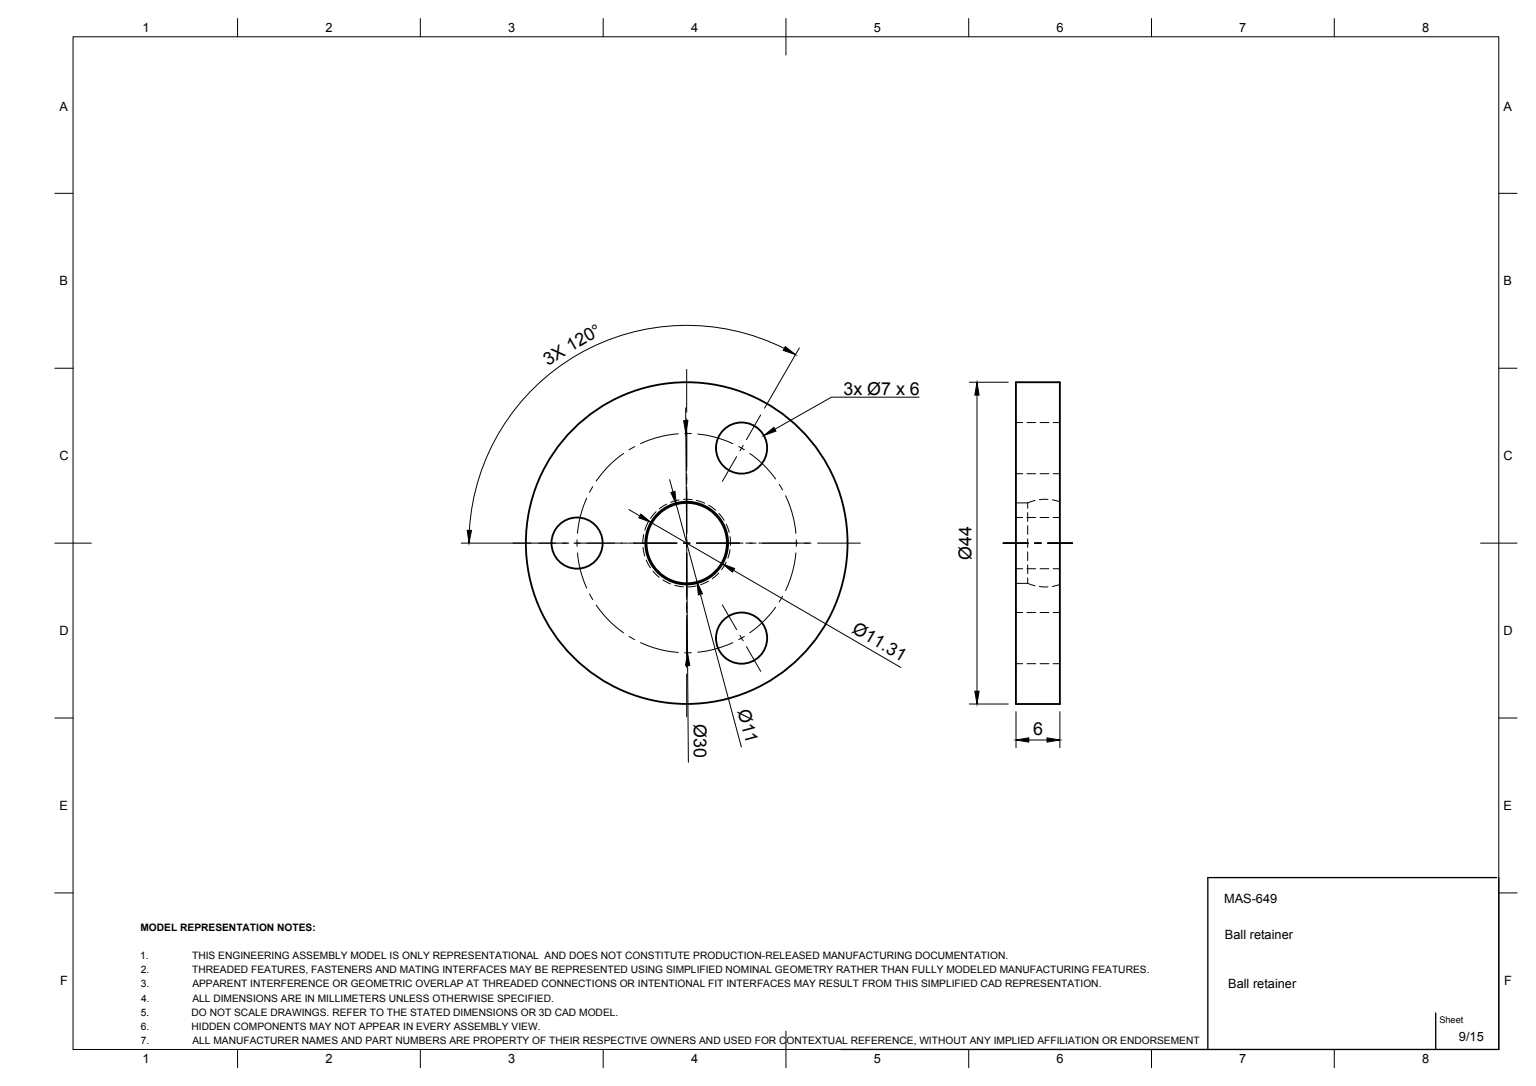
ISO-10303-21;
HEADER;
/* Generated by software containing ST-Developer
 * from STEP Tools, Inc. (www.steptools.com) 
 */

FILE_DESCRIPTION(
/* description */ ('Independent equipment support assembly with bolted 600 x 500 mm welde
d perimeter frame, four adjustable legs and swivel feet. Nominal overa
ll height 518 mm. No load rating assigned.'),
/* implementation_level */ '2;1');

FILE_NAME(
/* name */ 'Ball retainer.step',
/* time_stamp */ '2026-11-07T17:30:39-08:00',
/* author */ (''),
/* organization */ (''),
/* preprocessor_version */ 'ST-DEVELOPER v20.2',
/* originating_system */ 'Autodesk Translation Framework v15.17.0.0',
/* authorisation */ '');

FILE_SCHEMA (('AUTOMOTIVE_DESIGN { 1 0 10303 214 3 1 1 }'));
ENDSEC;

DATA;
#10=MECHANICAL_DESIGN_GEOMETRIC_PRESENTATION_REPRESENTATION('',(#2218),#63755);
#12=SPHERICAL_SURFACE('',#15242,6.);
#449=CIRCLE('',#15234,3.5);
#450=CIRCLE('',#15235,3.5);
#451=CIRCLE('',#15237,3.5);
#452=CIRCLE('',#15238,3.5);
#453=CIRCLE('',#15240,3.5);
#454=CIRCLE('',#15241,3.5);
#455=CIRCLE('',#15243,5.65685424949238);
#456=CIRCLE('',#15244,6.);
#457=CIRCLE('',#15245,5.5);
#458=CIRCLE('',#15247,5.5);
#459=CIRCLE('',#15249,22.);
#460=CIRCLE('',#15250,22.);
#1993=CYLINDRICAL_SURFACE('',#15233,3.5);
#1994=CYLINDRICAL_SURFACE('',#15236,3.5);
#1995=CYLINDRICAL_SURFACE('',#15239,3.5);
#1996=CYLINDRICAL_SURFACE('',#15246,5.5);
#1997=CYLINDRICAL_SURFACE('',#15248,22.);
#2186=SHAPE_REPRESENTATION_RELATIONSHIP('SRR','None',#63871,#2202);
#2202=ADVANCED_BREP_SHAPE_REPRESENTATION('',(#2234),#63749);
#2218=STYLED_ITEM('',(#63959),#2234);
#2234=MANIFOLD_SOLID_BREP('Body1',#14319);
#2285=FACE_BOUND('',#3650,.T.);
#2286=FACE_BOUND('',#3651,.T.);
#2287=FACE_BOUND('',#3652,.T.);
#2288=FACE_BOUND('',#3653,.T.);
#2289=FACE_BOUND('',#3655,.T.);
#2290=FACE_BOUND('',#3656,.T.);
#2291=FACE_BOUND('',#3657,.T.);
#2292=FACE_BOUND('',#3658,.T.);
#2838=FACE_OUTER_BOUND('',#3643,.T.);
#2839=FACE_OUTER_BOUND('',#3644,.T.);
#2840=FACE_OUTER_BOUND('',#3645,.T.);
#2841=FACE_OUTER_BOUND('',#3646,.T.);
#2842=FACE_OUTER_BOUND('',#3647,.T.);
#2843=FACE_OUTER_BOUND('',#3648,.T.);
#2844=FACE_OUTER_BOUND('',#3649,.T.);
#2845=FACE_OUTER_BOUND('',#3654,.T.);
#3643=EDGE_LOOP('',(#12155,#12156,#12157,#12158));
#3644=EDGE_LOOP('',(#12159,#12160,#12161,#12162));
#3645=EDGE_LOOP('',(#12163,#12164,#12165,#12166));
#3646=EDGE_LOOP('',(#12167,#12168,#12169,#12170));
#3647=EDGE_LOOP('',(#12171,#12172,#12173,#12174));
#3648=EDGE_LOOP('',(#12175,#12176,#12177,#12178));
#3649=EDGE_LOOP('',(#12179));
#3650=EDGE_LOOP('',(#12180));
#3651=EDGE_LOOP('',(#12181));
#3652=EDGE_LOOP('',(#12182));
#3653=EDGE_LOOP('',(#12183));
#3654=EDGE_LOOP('',(#12184));
#3655=EDGE_LOOP('',(#12185));
#3656=EDGE_LOOP('',(#12186));
#3657=EDGE_LOOP('',(#12187));
#3658=EDGE_LOOP('',(#12188));
#4490=LINE('',#51513,#5326);
#4491=LINE('',#51519,#5327);
#4492=LINE('',#51525,#5328);
#4493=LINE('',#51536,#5329);
#4494=LINE('',#51541,#5330);
#5326=VECTOR('',#17585,3.5);
#5327=VECTOR('',#17592,3.5);
#5328=VECTOR('',#17599,3.5);
#5329=VECTOR('',#17614,5.5);
#5330=VECTOR('',#17619,22.);
#6568=VERTEX_POINT('',#51510);
#6569=VERTEX_POINT('',#51512);
#6570=VERTEX_POINT('',#51516);
#6571=VERTEX_POINT('',#51518);
#6572=VERTEX_POINT('',#51522);
#6573=VERTEX_POINT('',#51524);
#6574=VERTEX_POINT('',#51528);
#6575=VERTEX_POINT('',#51530);
#6576=VERTEX_POINT('',#51534);
#6577=VERTEX_POINT('',#51538);
#6578=VERTEX_POINT('',#51540);
#8500=EDGE_CURVE('',#6568,#6568,#449,.T.);
#8501=EDGE_CURVE('',#6568,#6569,#4490,.T.);
#8502=EDGE_CURVE('',#6569,#6569,#450,.T.);
#8503=EDGE_CURVE('',#6570,#6570,#451,.T.);
#8504=EDGE_CURVE('',#6570,#6571,#4491,.T.);
#8505=EDGE_CURVE('',#6571,#6571,#452,.T.);
#8506=EDGE_CURVE('',#6572,#6572,#453,.T.);
#8507=EDGE_CURVE('',#6572,#6573,#4492,.T.);
#8508=EDGE_CURVE('',#6573,#6573,#454,.T.);
#8509=EDGE_CURVE('',#6574,#6574,#455,.T.);
#8510=EDGE_CURVE('',#6574,#6575,#456,.T.);
#8511=EDGE_CURVE('',#6575,#6575,#457,.T.);
#8512=EDGE_CURVE('',#6576,#6576,#458,.T.);
#8513=EDGE_CURVE('',#6576,#6575,#4493,.T.);
#8514=EDGE_CURVE('',#6577,#6577,#459,.T.);
#8515=EDGE_CURVE('',#6577,#6578,#4494,.T.);
#8516=EDGE_CURVE('',#6578,#6578,#460,.T.);
#12155=ORIENTED_EDGE('',*,*,#8500,.F.);
#12156=ORIENTED_EDGE('',*,*,#8501,.T.);
#12157=ORIENTED_EDGE('',*,*,#8502,.F.);
#12158=ORIENTED_EDGE('',*,*,#8501,.F.);
#12159=ORIENTED_EDGE('',*,*,#8503,.F.);
#12160=ORIENTED_EDGE('',*,*,#8504,.T.);
#12161=ORIENTED_EDGE('',*,*,#8505,.F.);
#12162=ORIENTED_EDGE('',*,*,#8504,.F.);
#12163=ORIENTED_EDGE('',*,*,#8506,.F.);
#12164=ORIENTED_EDGE('',*,*,#8507,.T.);
#12165=ORIENTED_EDGE('',*,*,#8508,.F.);
#12166=ORIENTED_EDGE('',*,*,#8507,.F.);
#12167=ORIENTED_EDGE('',*,*,#8509,.F.);
#12168=ORIENTED_EDGE('',*,*,#8510,.T.);
#12169=ORIENTED_EDGE('',*,*,#8511,.F.);
#12170=ORIENTED_EDGE('',*,*,#8510,.F.);
#12171=ORIENTED_EDGE('',*,*,#8512,.F.);
#12172=ORIENTED_EDGE('',*,*,#8513,.T.);
#12173=ORIENTED_EDGE('',*,*,#8511,.T.);
#12174=ORIENTED_EDGE('',*,*,#8513,.F.);
#12175=ORIENTED_EDGE('',*,*,#8514,.F.);
#12176=ORIENTED_EDGE('',*,*,#8515,.T.);
#12177=ORIENTED_EDGE('',*,*,#8516,.T.);
#12178=ORIENTED_EDGE('',*,*,#8515,.F.);
#12179=ORIENTED_EDGE('',*,*,#8514,.T.);
#12180=ORIENTED_EDGE('',*,*,#8500,.T.);
#12181=ORIENTED_EDGE('',*,*,#8503,.T.);
#12182=ORIENTED_EDGE('',*,*,#8506,.T.);
#12183=ORIENTED_EDGE('',*,*,#8512,.T.);
#12184=ORIENTED_EDGE('',*,*,#8516,.F.);
#12185=ORIENTED_EDGE('',*,*,#8502,.T.);
#12186=ORIENTED_EDGE('',*,*,#8505,.T.);
#12187=ORIENTED_EDGE('',*,*,#8508,.T.);
#12188=ORIENTED_EDGE('',*,*,#8509,.T.);
#13516=PLANE('',#15251);
#13517=PLANE('',#15252);
#14084=ADVANCED_FACE('',(#2838),#1993,.F.);
#14085=ADVANCED_FACE('',(#2839),#1994,.F.);
#14086=ADVANCED_FACE('',(#2840),#1995,.F.);
#14087=ADVANCED_FACE('',(#2841),#12,.F.);
#14088=ADVANCED_FACE('',(#2842),#1996,.F.);
#14089=ADVANCED_FACE('',(#2843),#1997,.T.);
#14090=ADVANCED_FACE('',(#2844,#2285,#2286,#2287,#2288),#13516,.T.);
#14091=ADVANCED_FACE('',(#2845,#2289,#2290,#2291,#2292),#13517,.F.);
#14319=CLOSED_SHELL('',(#14084,#14085,#14086,#14087,#14088,#14089,#14090,
#14091));
#15232=AXIS2_PLACEMENT_3D('',#51508,#17579,#17580);
#15233=AXIS2_PLACEMENT_3D('',#51509,#17581,#17582);
#15234=AXIS2_PLACEMENT_3D('',#51511,#17583,#17584);
#15235=AXIS2_PLACEMENT_3D('',#51514,#17586,#17587);
#15236=AXIS2_PLACEMENT_3D('',#51515,#17588,#17589);
#15237=AXIS2_PLACEMENT_3D('',#51517,#17590,#17591);
#15238=AXIS2_PLACEMENT_3D('',#51520,#17593,#17594);
#15239=AXIS2_PLACEMENT_3D('',#51521,#17595,#17596);
#15240=AXIS2_PLACEMENT_3D('',#51523,#17597,#17598);
#15241=AXIS2_PLACEMENT_3D('',#51526,#17600,#17601);
#15242=AXIS2_PLACEMENT_3D('',#51527,#17602,#17603);
#15243=AXIS2_PLACEMENT_3D('',#51529,#17604,#17605);
#15244=AXIS2_PLACEMENT_3D('',#51531,#17606,#17607);
#15245=AXIS2_PLACEMENT_3D('',#51532,#17608,#17609);
#15246=AXIS2_PLACEMENT_3D('',#51533,#17610,#17611);
#15247=AXIS2_PLACEMENT_3D('',#51535,#17612,#17613);
#15248=AXIS2_PLACEMENT_3D('',#51537,#17615,#17616);
#15249=AXIS2_PLACEMENT_3D('',#51539,#17617,#17618);
#15250=AXIS2_PLACEMENT_3D('',#51542,#17620,#17621);
#15251=AXIS2_PLACEMENT_3D('',#51543,#17622,#17623);
#15252=AXIS2_PLACEMENT_3D('',#51544,#17624,#17625);
#17579=DIRECTION('axis',(0.,0.,1.));
#17580=DIRECTION('refdir',(1.,0.,0.));
#17581=DIRECTION('center_axis',(0.,0.,-1.));
#17582=DIRECTION('ref_axis',(1.,0.,0.));
#17583=DIRECTION('center_axis',(0.,0.,-1.));
#17584=DIRECTION('ref_axis',(1.,0.,0.));
#17585=DIRECTION('',(0.,0.,-1.));
#17586=DIRECTION('center_axis',(0.,0.,1.));
#17587=DIRECTION('ref_axis',(1.,0.,0.));
#17588=DIRECTION('center_axis',(0.,0.,-1.));
#17589=DIRECTION('ref_axis',(1.,0.,0.));
#17590=DIRECTION('center_axis',(0.,0.,-1.));
#17591=DIRECTION('ref_axis',(1.,0.,0.));
#17592=DIRECTION('',(0.,0.,-1.));
#17593=DIRECTION('center_axis',(0.,0.,1.));
#17594=DIRECTION('ref_axis',(1.,0.,0.));
#17595=DIRECTION('center_axis',(0.,0.,-1.));
#17596=DIRECTION('ref_axis',(1.,0.,0.));
#17597=DIRECTION('center_axis',(0.,0.,-1.));
#17598=DIRECTION('ref_axis',(1.,0.,0.));
#17599=DIRECTION('',(0.,0.,-1.));
#17600=DIRECTION('center_axis',(0.,0.,1.));
#17601=DIRECTION('ref_axis',(1.,0.,0.));
#17602=DIRECTION('center_axis',(6.12323399573677E-17,0.,1.));
#17603=DIRECTION('ref_axis',(1.,0.,0.));
#17604=DIRECTION('center_axis',(0.,0.,1.));
#17605=DIRECTION('ref_axis',(0.,-1.,0.));
#17606=DIRECTION('center_axis',(-1.22464679914735E-16,1.,0.));
#17607=DIRECTION('ref_axis',(-1.,-1.22464679914735E-16,0.));
#17608=DIRECTION('center_axis',(0.,0.,-1.));
#17609=DIRECTION('ref_axis',(1.,0.,0.));
#17610=DIRECTION('center_axis',(0.,0.,1.));
#17611=DIRECTION('ref_axis',(1.,0.,0.));
#17612=DIRECTION('center_axis',(0.,0.,-1.));
#17613=DIRECTION('ref_axis',(1.,0.,0.));
#17614=DIRECTION('',(0.,0.,-1.));
#17615=DIRECTION('center_axis',(0.,0.,1.));
#17616=DIRECTION('ref_axis',(1.,0.,0.));
#17617=DIRECTION('center_axis',(0.,0.,1.));
#17618=DIRECTION('ref_axis',(1.,0.,0.));
#17619=DIRECTION('',(0.,0.,-1.));
#17620=DIRECTION('center_axis',(0.,0.,1.));
#17621=DIRECTION('ref_axis',(1.,0.,0.));
#17622=DIRECTION('center_axis',(0.,0.,1.));
#17623=DIRECTION('ref_axis',(1.,0.,0.));
#17624=DIRECTION('center_axis',(0.,0.,1.));
#17625=DIRECTION('ref_axis',(1.,0.,0.));
#51508=CARTESIAN_POINT('',(0.,0.,0.));
#51509=CARTESIAN_POINT('Origin',(-7.5,12.9903810567666,15.));
#51510=CARTESIAN_POINT('',(-11.,12.9903810567666,18.));
#51511=CARTESIAN_POINT('Origin',(-7.5,12.9903810567666,18.));
#51512=CARTESIAN_POINT('',(-11.,12.9903810567666,12.));
#51513=CARTESIAN_POINT('',(-11.,12.9903810567666,15.));
#51514=CARTESIAN_POINT('Origin',(-7.5,12.9903810567666,12.));
#51515=CARTESIAN_POINT('Origin',(15.,0.,15.));
#51516=CARTESIAN_POINT('',(11.5,4.28626379701574E-16,18.));
#51517=CARTESIAN_POINT('Origin',(15.,0.,18.));
#51518=CARTESIAN_POINT('',(11.5,4.28626379701574E-16,12.));
#51519=CARTESIAN_POINT('',(11.5,4.28626379701574E-16,15.));
#51520=CARTESIAN_POINT('Origin',(15.,0.,12.));
#51521=CARTESIAN_POINT('Origin',(-7.50000000000001,-12.9903810567666,15.));
#51522=CARTESIAN_POINT('',(-11.,-12.9903810567666,18.));
#51523=CARTESIAN_POINT('Origin',(-7.50000000000001,-12.9903810567666,18.));
#51524=CARTESIAN_POINT('',(-11.,-12.9903810567666,12.));
#51525=CARTESIAN_POINT('',(-11.,-12.9903810567666,15.));
#51526=CARTESIAN_POINT('Origin',(-7.50000000000001,-12.9903810567666,12.));
#51527=CARTESIAN_POINT('Origin',(5.55111512312578E-16,0.,14.));
#51528=CARTESIAN_POINT('',(-5.65685424949238,-6.92764844988394E-16,12.));
#51529=CARTESIAN_POINT('Origin',(5.55111512312578E-16,0.,12.));
#51530=CARTESIAN_POINT('',(-5.5,6.73555739531044E-16,16.3979157616564));
#51531=CARTESIAN_POINT('Origin',(5.55111512312578E-16,0.,14.));
#51532=CARTESIAN_POINT('Origin',(0.,0.,16.3979157616564));
#51533=CARTESIAN_POINT('Origin',(0.,0.,12.));
#51534=CARTESIAN_POINT('',(-5.5,-6.73555739531044E-16,18.));
#51535=CARTESIAN_POINT('Origin',(0.,0.,18.));
#51536=CARTESIAN_POINT('',(-5.5,-6.73555739531044E-16,12.));
#51537=CARTESIAN_POINT('Origin',(0.,0.,12.));
#51538=CARTESIAN_POINT('',(-22.,-2.69422295812418E-15,18.));
#51539=CARTESIAN_POINT('Origin',(0.,0.,18.));
#51540=CARTESIAN_POINT('',(-22.,-2.69422295812418E-15,12.));
#51541=CARTESIAN_POINT('',(-22.,-2.69422295812418E-15,12.));
#51542=CARTESIAN_POINT('Origin',(0.,0.,12.));
#51543=CARTESIAN_POINT('Origin',(0.,0.,18.));
#51544=CARTESIAN_POINT('Origin',(0.,0.,12.));
#63729=UNCERTAINTY_MEASURE_WITH_UNIT(LENGTH_MEASURE(0.01),#63756,
'DISTANCE_ACCURACY_VALUE',
'Maximum model space distance between geometric entities at asserted c
onnectivities');
#63735=UNCERTAINTY_MEASURE_WITH_UNIT(LENGTH_MEASURE(0.01),#63756,
'DISTANCE_ACCURACY_VALUE',
'Maximum model space distance between geometric entities at asserted c
onnectivities');
#63749=(
GEOMETRIC_REPRESENTATION_CONTEXT(3)
GLOBAL_UNCERTAINTY_ASSIGNED_CONTEXT((#63729))
GLOBAL_UNIT_ASSIGNED_CONTEXT((#63756,#63758,#63759))
REPRESENTATION_CONTEXT('','3D')
);
#63755=(
GEOMETRIC_REPRESENTATION_CONTEXT(3)
GLOBAL_UNCERTAINTY_ASSIGNED_CONTEXT((#63735))
GLOBAL_UNIT_ASSIGNED_CONTEXT((#63756,#63758,#63759))
REPRESENTATION_CONTEXT('','3D')
);
#63756=(
LENGTH_UNIT()
NAMED_UNIT(*)
SI_UNIT(.MILLI.,.METRE.)
);
#63758=(
NAMED_UNIT(*)
PLANE_ANGLE_UNIT()
SI_UNIT($,.RADIAN.)
);
#63759=(
NAMED_UNIT(*)
SI_UNIT($,.STERADIAN.)
SOLID_ANGLE_UNIT()
);
#63773=SHAPE_DEFINITION_REPRESENTATION(#63832,#63871);
#63832=PRODUCT_DEFINITION_SHAPE('',$,#63891);
#63871=SHAPE_REPRESENTATION('',(#15232),#63749);
#63877=PRODUCT_DEFINITION_CONTEXT('part definition',#63936,'design');
#63891=PRODUCT_DEFINITION('Ball retainer','Ball retainer',#63910,#63877);
#63910=PRODUCT_DEFINITION_FORMATION('',$,#63951);
#63936=APPLICATION_CONTEXT(
'Core Data for Automotive Mechanical Design Process');
#63937=PRODUCT_CONTEXT('part definition',#63936,'mechanical');
#63951=PRODUCT('Ball retainer','Ball retainer',$,(#63937));
#63959=PRESENTATION_STYLE_ASSIGNMENT((#63966));
#63966=SURFACE_STYLE_USAGE(.BOTH.,#63973);
#63973=SURFACE_SIDE_STYLE('',(#63980));
#63980=SURFACE_STYLE_FILL_AREA(#63987);
#63987=FILL_AREA_STYLE('Sky blue',(#63994));
#63994=FILL_AREA_STYLE_COLOUR('Sky blue',#64001);
#64001=COLOUR_RGB('Sky blue',0.317647058823529,0.686274509803922,0.890196078431372);
ENDSEC;
END-ISO-10303-21;
